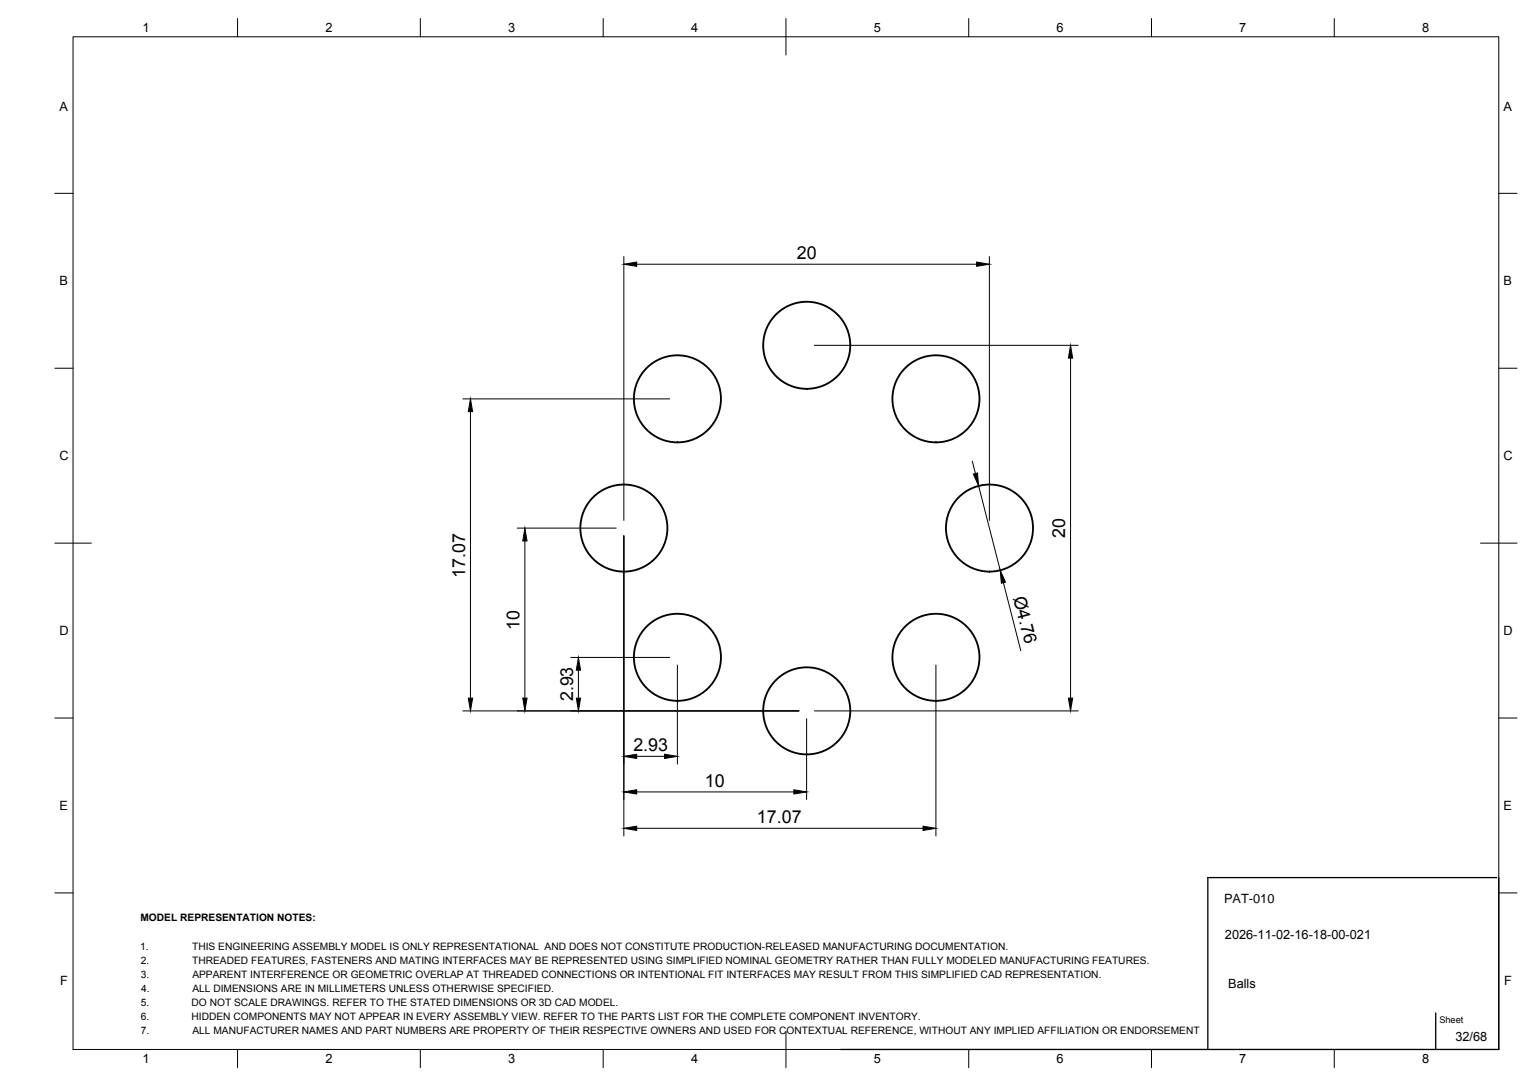
ISO-10303-21;
HEADER;
/* Generated by software containing ST-Developer
 * from STEP Tools, Inc. (www.steptools.com) 
 */

FILE_DESCRIPTION(
/* description */ ('Belt conveyor head drive unit'),
/* implementation_level */ '2;1');

FILE_NAME(
/* name */ 'Balls.step',
/* time_stamp */ '2026-10-28T03:26:19-07:00',
/* author */ (''),
/* organization */ (''),
/* preprocessor_version */ 'ST-DEVELOPER v20.2',
/* originating_system */ 'Autodesk Translation Framework v15.17.0.0',
/* authorisation */ '');

FILE_SCHEMA (('AUTOMOTIVE_DESIGN { 1 0 10303 214 3 1 1 }'));
ENDSEC;

DATA;
#10=MECHANICAL_DESIGN_GEOMETRIC_PRESENTATION_REPRESENTATION('',(#876,#877,#878,#879,#880,#881,#882,#883),#27069);
#645=SPHERICAL_SURFACE('',#15231,0.23815);
#646=SPHERICAL_SURFACE('',#15233,0.23815);
#647=SPHERICAL_SURFACE('',#15235,0.23815);
#648=SPHERICAL_SURFACE('',#15237,0.23815);
#649=SPHERICAL_SURFACE('',#15239,0.23815);
#650=SPHERICAL_SURFACE('',#15241,0.23815);
#651=SPHERICAL_SURFACE('',#15243,0.23815);
#652=SPHERICAL_SURFACE('',#15245,0.23815);
#738=SHAPE_REPRESENTATION_RELATIONSHIP('SRR','None',#27383,#807);
#807=ADVANCED_BREP_SHAPE_REPRESENTATION('',(#961,#962,#963,#964,#965,#966,
#967,#968),#27025);
#876=STYLED_ITEM('',(#27797),#961);
#877=STYLED_ITEM('',(#27797),#962);
#878=STYLED_ITEM('',(#27797),#963);
#879=STYLED_ITEM('',(#27797),#964);
#880=STYLED_ITEM('',(#27797),#965);
#881=STYLED_ITEM('',(#27797),#966);
#882=STYLED_ITEM('',(#27797),#967);
#883=STYLED_ITEM('',(#27797),#968);
#961=MANIFOLD_SOLID_BREP('Body1',#13741);
#962=MANIFOLD_SOLID_BREP('Body2',#13742);
#963=MANIFOLD_SOLID_BREP('Body3',#13743);
#964=MANIFOLD_SOLID_BREP('Body4',#13744);
#965=MANIFOLD_SOLID_BREP('Body5',#13745);
#966=MANIFOLD_SOLID_BREP('Body6',#13746);
#967=MANIFOLD_SOLID_BREP('Body7',#13747);
#968=MANIFOLD_SOLID_BREP('Body8',#13748);
#1951=FACE_OUTER_BOUND('',#2894,.T.);
#1952=FACE_OUTER_BOUND('',#2895,.T.);
#1953=FACE_OUTER_BOUND('',#2896,.T.);
#1954=FACE_OUTER_BOUND('',#2897,.T.);
#1955=FACE_OUTER_BOUND('',#2898,.T.);
#1956=FACE_OUTER_BOUND('',#2899,.T.);
#1957=FACE_OUTER_BOUND('',#2900,.T.);
#1958=FACE_OUTER_BOUND('',#2901,.T.);
#2894=EDGE_LOOP('',(#10336,#10337));
#2895=EDGE_LOOP('',(#10338,#10339));
#2896=EDGE_LOOP('',(#10340,#10341));
#2897=EDGE_LOOP('',(#10342,#10343));
#2898=EDGE_LOOP('',(#10344,#10345));
#2899=EDGE_LOOP('',(#10346,#10347));
#2900=EDGE_LOOP('',(#10348,#10349));
#2901=EDGE_LOOP('',(#10350,#10351));
#5400=CIRCLE('',#15232,0.23815);
#5401=CIRCLE('',#15234,0.23815);
#5402=CIRCLE('',#15236,0.23815);
#5403=CIRCLE('',#15238,0.23815);
#5404=CIRCLE('',#15240,0.23815);
#5405=CIRCLE('',#15242,0.23815);
#5406=CIRCLE('',#15244,0.23815);
#5407=CIRCLE('',#15246,0.23815);
#6411=VERTEX_POINT('',#22469);
#6412=VERTEX_POINT('',#22470);
#6413=VERTEX_POINT('',#22473);
#6414=VERTEX_POINT('',#22474);
#6415=VERTEX_POINT('',#22477);
#6416=VERTEX_POINT('',#22478);
#6417=VERTEX_POINT('',#22481);
#6418=VERTEX_POINT('',#22482);
#6419=VERTEX_POINT('',#22485);
#6420=VERTEX_POINT('',#22486);
#6421=VERTEX_POINT('',#22489);
#6422=VERTEX_POINT('',#22490);
#6423=VERTEX_POINT('',#22493);
#6424=VERTEX_POINT('',#22494);
#6425=VERTEX_POINT('',#22497);
#6426=VERTEX_POINT('',#22498);
#7860=EDGE_CURVE('',#6411,#6412,#5400,.T.);
#7861=EDGE_CURVE('',#6413,#6414,#5401,.T.);
#7862=EDGE_CURVE('',#6415,#6416,#5402,.T.);
#7863=EDGE_CURVE('',#6417,#6418,#5403,.T.);
#7864=EDGE_CURVE('',#6419,#6420,#5404,.T.);
#7865=EDGE_CURVE('',#6421,#6422,#5405,.T.);
#7866=EDGE_CURVE('',#6423,#6424,#5406,.T.);
#7867=EDGE_CURVE('',#6425,#6426,#5407,.T.);
#10336=ORIENTED_EDGE('',*,*,#7860,.T.);
#10337=ORIENTED_EDGE('',*,*,#7860,.F.);
#10338=ORIENTED_EDGE('',*,*,#7861,.T.);
#10339=ORIENTED_EDGE('',*,*,#7861,.F.);
#10340=ORIENTED_EDGE('',*,*,#7862,.T.);
#10341=ORIENTED_EDGE('',*,*,#7862,.F.);
#10342=ORIENTED_EDGE('',*,*,#7863,.T.);
#10343=ORIENTED_EDGE('',*,*,#7863,.F.);
#10344=ORIENTED_EDGE('',*,*,#7864,.T.);
#10345=ORIENTED_EDGE('',*,*,#7864,.F.);
#10346=ORIENTED_EDGE('',*,*,#7865,.T.);
#10347=ORIENTED_EDGE('',*,*,#7865,.F.);
#10348=ORIENTED_EDGE('',*,*,#7866,.T.);
#10349=ORIENTED_EDGE('',*,*,#7866,.F.);
#10350=ORIENTED_EDGE('',*,*,#7867,.T.);
#10351=ORIENTED_EDGE('',*,*,#7867,.F.);
#13230=ADVANCED_FACE('',(#1951),#645,.T.);
#13231=ADVANCED_FACE('',(#1952),#646,.T.);
#13232=ADVANCED_FACE('',(#1953),#647,.T.);
#13233=ADVANCED_FACE('',(#1954),#648,.T.);
#13234=ADVANCED_FACE('',(#1955),#649,.T.);
#13235=ADVANCED_FACE('',(#1956),#650,.T.);
#13236=ADVANCED_FACE('',(#1957),#651,.T.);
#13237=ADVANCED_FACE('',(#1958),#652,.T.);
#13741=CLOSED_SHELL('',(#13230));
#13742=CLOSED_SHELL('',(#13231));
#13743=CLOSED_SHELL('',(#13232));
#13744=CLOSED_SHELL('',(#13233));
#13745=CLOSED_SHELL('',(#13234));
#13746=CLOSED_SHELL('',(#13235));
#13747=CLOSED_SHELL('',(#13236));
#13748=CLOSED_SHELL('',(#13237));
#15230=AXIS2_PLACEMENT_3D('',#22467,#18141,#18142);
#15231=AXIS2_PLACEMENT_3D('',#22468,#18143,#18144);
#15232=AXIS2_PLACEMENT_3D('',#22471,#18145,#18146);
#15233=AXIS2_PLACEMENT_3D('',#22472,#18147,#18148);
#15234=AXIS2_PLACEMENT_3D('',#22475,#18149,#18150);
#15235=AXIS2_PLACEMENT_3D('',#22476,#18151,#18152);
#15236=AXIS2_PLACEMENT_3D('',#22479,#18153,#18154);
#15237=AXIS2_PLACEMENT_3D('',#22480,#18155,#18156);
#15238=AXIS2_PLACEMENT_3D('',#22483,#18157,#18158);
#15239=AXIS2_PLACEMENT_3D('',#22484,#18159,#18160);
#15240=AXIS2_PLACEMENT_3D('',#22487,#18161,#18162);
#15241=AXIS2_PLACEMENT_3D('',#22488,#18163,#18164);
#15242=AXIS2_PLACEMENT_3D('',#22491,#18165,#18166);
#15243=AXIS2_PLACEMENT_3D('',#22492,#18167,#18168);
#15244=AXIS2_PLACEMENT_3D('',#22495,#18169,#18170);
#15245=AXIS2_PLACEMENT_3D('',#22496,#18171,#18172);
#15246=AXIS2_PLACEMENT_3D('',#22499,#18173,#18174);
#18141=DIRECTION('axis',(0.,0.,1.));
#18142=DIRECTION('refdir',(1.,0.,0.));
#18143=DIRECTION('center_axis',(0.,0.,1.));
#18144=DIRECTION('ref_axis',(1.,0.,0.));
#18145=DIRECTION('center_axis',(1.22464679914735E-16,-1.,0.));
#18146=DIRECTION('ref_axis',(-1.,-1.22464679914735E-16,0.));
#18147=DIRECTION('center_axis',(0.707106781186548,0.,0.707106781186548));
#18148=DIRECTION('ref_axis',(0.707106781186548,0.,-0.707106781186548));
#18149=DIRECTION('center_axis',(8.65956056235494E-17,-1.,-8.65956056235493E-17));
#18150=DIRECTION('ref_axis',(-0.707106781186547,-1.22464679914735E-16,0.707106781186547));
#18151=DIRECTION('center_axis',(1.,0.,0.));
#18152=DIRECTION('ref_axis',(6.12323399573676E-17,0.,-1.));
#18153=DIRECTION('center_axis',(7.49879891330929E-33,-1.,-1.22464679914735E-16));
#18154=DIRECTION('ref_axis',(-6.12323399573676E-17,-1.22464679914735E-16,
1.));
#18155=DIRECTION('center_axis',(0.707106781186548,0.,-0.707106781186548));
#18156=DIRECTION('ref_axis',(-0.707106781186548,0.,-0.707106781186548));
#18157=DIRECTION('center_axis',(-8.65956056235493E-17,-1.,-8.65956056235494E-17));
#18158=DIRECTION('ref_axis',(0.707106781186547,-1.22464679914735E-16,0.707106781186547));
#18159=DIRECTION('center_axis',(0.,0.,-1.));
#18160=DIRECTION('ref_axis',(-1.,0.,-1.22464679914735E-16));
#18161=DIRECTION('center_axis',(-1.22464679914735E-16,-1.,-1.49975978266186E-32));
#18162=DIRECTION('ref_axis',(1.,-1.22464679914735E-16,1.22464679914735E-16));
#18163=DIRECTION('center_axis',(-0.707106781186547,0.,-0.707106781186548));
#18164=DIRECTION('ref_axis',(-0.707106781186548,0.,0.707106781186547));
#18165=DIRECTION('center_axis',(-8.65956056235493E-17,-1.,8.65956056235493E-17));
#18166=DIRECTION('ref_axis',(0.707106781186548,-1.22464679914735E-16,-0.707106781186547));
#18167=DIRECTION('center_axis',(-1.,0.,0.));
#18168=DIRECTION('ref_axis',(-1.83697019872103E-16,0.,1.));
#18169=DIRECTION('center_axis',(-2.24963967399279E-32,-1.,1.22464679914735E-16));
#18170=DIRECTION('ref_axis',(1.83697019872103E-16,-1.22464679914735E-16,
-1.));
#18171=DIRECTION('center_axis',(-0.707106781186548,0.,0.707106781186548));
#18172=DIRECTION('ref_axis',(0.707106781186547,0.,0.707106781186548));
#18173=DIRECTION('center_axis',(8.65956056235493E-17,-1.,8.65956056235493E-17));
#18174=DIRECTION('ref_axis',(-0.707106781186547,-1.22464679914735E-16,-0.707106781186548));
#22467=CARTESIAN_POINT('',(0.,0.,0.));
#22468=CARTESIAN_POINT('Origin',(1.,0.,0.));
#22469=CARTESIAN_POINT('',(1.,-1.78583896120461E-33,0.23815));
#22470=CARTESIAN_POINT('',(1.,-1.78583896120461E-33,-0.23815));
#22471=CARTESIAN_POINT('Origin',(1.,0.,0.));
#22472=CARTESIAN_POINT('Origin',(0.707106781186548,0.,-0.707106781186547));
#22473=CARTESIAN_POINT('',(0.875504261126124,-1.78583896120461E-33,-0.538709301246971));
#22474=CARTESIAN_POINT('',(0.538709301246971,-1.78583896120461E-33,-0.875504261126124));
#22475=CARTESIAN_POINT('Origin',(0.707106781186548,0.,-0.707106781186547));
#22476=CARTESIAN_POINT('Origin',(6.12323399573677E-17,0.,-1.));
#22477=CARTESIAN_POINT('',(0.23815,-1.78583896120461E-33,-1.));
#22478=CARTESIAN_POINT('',(-0.23815,-1.78583896120461E-33,-1.));
#22479=CARTESIAN_POINT('Origin',(6.12323399573677E-17,0.,-1.));
#22480=CARTESIAN_POINT('Origin',(-0.707106781186547,0.,-0.707106781186548));
#22481=CARTESIAN_POINT('',(-0.538709301246971,-1.78583896120461E-33,-0.875504261126124));
#22482=CARTESIAN_POINT('',(-0.875504261126124,-1.78583896120461E-33,-0.538709301246971));
#22483=CARTESIAN_POINT('Origin',(-0.707106781186547,0.,-0.707106781186548));
#22484=CARTESIAN_POINT('Origin',(-1.,0.,-1.22464679914735E-16));
#22485=CARTESIAN_POINT('',(-1.,-1.78583896120461E-33,-0.23815));
#22486=CARTESIAN_POINT('',(-1.,-1.78583896120461E-33,0.23815));
#22487=CARTESIAN_POINT('Origin',(-1.,0.,-1.22464679914735E-16));
#22488=CARTESIAN_POINT('Origin',(-0.707106781186548,0.,0.707106781186547));
#22489=CARTESIAN_POINT('',(-0.875504261126124,-7.94881478324376E-33,0.538709301246971));
#22490=CARTESIAN_POINT('',(-0.538709301246971,4.37713686083455E-33,0.875504261126124));
#22491=CARTESIAN_POINT('Origin',(-0.707106781186548,0.,0.707106781186547));
#22492=CARTESIAN_POINT('Origin',(-1.83697019872103E-16,0.,1.));
#22493=CARTESIAN_POINT('',(-0.23815,-1.78583896120461E-33,1.));
#22494=CARTESIAN_POINT('',(0.23815,-1.78583896120461E-33,1.));
#22495=CARTESIAN_POINT('Origin',(-1.83697019872103E-16,0.,1.));
#22496=CARTESIAN_POINT('Origin',(0.707106781186547,0.,0.707106781186548));
#22497=CARTESIAN_POINT('',(0.538709301246971,-4.86732687222419E-33,0.875504261126124));
#22498=CARTESIAN_POINT('',(0.875504261126124,1.29564894981497E-33,0.538709301246971));
#22499=CARTESIAN_POINT('Origin',(0.707106781186547,0.,0.707106781186548));
#26948=UNCERTAINTY_MEASURE_WITH_UNIT(LENGTH_MEASURE(0.001),#27070,
'DISTANCE_ACCURACY_VALUE',
'Maximum model space distance between geometric entities at asserted c
onnectivities');
#26992=UNCERTAINTY_MEASURE_WITH_UNIT(LENGTH_MEASURE(0.001),#27070,
'DISTANCE_ACCURACY_VALUE',
'Maximum model space distance between geometric entities at asserted c
onnectivities');
#27025=(
GEOMETRIC_REPRESENTATION_CONTEXT(3)
GLOBAL_UNCERTAINTY_ASSIGNED_CONTEXT((#26948))
GLOBAL_UNIT_ASSIGNED_CONTEXT((#27070,#27072,#27073))
REPRESENTATION_CONTEXT('','3D')
);
#27069=(
GEOMETRIC_REPRESENTATION_CONTEXT(3)
GLOBAL_UNCERTAINTY_ASSIGNED_CONTEXT((#26992))
GLOBAL_UNIT_ASSIGNED_CONTEXT((#27070,#27072,#27073))
REPRESENTATION_CONTEXT('','3D')
);
#27070=(
LENGTH_UNIT()
NAMED_UNIT(*)
SI_UNIT(.CENTI.,.METRE.)
);
#27072=(
NAMED_UNIT(*)
PLANE_ANGLE_UNIT()
SI_UNIT($,.RADIAN.)
);
#27073=(
NAMED_UNIT(*)
SI_UNIT($,.STERADIAN.)
SOLID_ANGLE_UNIT()
);
#27106=SHAPE_DEFINITION_REPRESENTATION(#27182,#27383);
#27182=PRODUCT_DEFINITION_SHAPE('',$,#27460);
#27383=SHAPE_REPRESENTATION('',(#15230),#27025);
#27427=PRODUCT_DEFINITION_CONTEXT('part definition',#27657,'design');
#27460=PRODUCT_DEFINITION('Balls','Balls',#27536,#27427);
#27536=PRODUCT_DEFINITION_FORMATION('',$,#27691);
#27657=APPLICATION_CONTEXT(
'Core Data for Automotive Mechanical Design Process');
#27658=PRODUCT_CONTEXT('part definition',#27657,'mechanical');
#27691=PRODUCT('Balls','Balls','Balls',(#27658));
#27791=COLOUR_RGB('Grey',0.48,0.52,0.57);
#27792=FILL_AREA_STYLE_COLOUR('',#27791);
#27793=FILL_AREA_STYLE('',(#27792));
#27794=SURFACE_STYLE_FILL_AREA(#27793);
#27795=SURFACE_SIDE_STYLE('',(#27794));
#27796=SURFACE_STYLE_USAGE(.BOTH.,#27795);
#27797=PRESENTATION_STYLE_ASSIGNMENT((#27796));
ENDSEC;
END-ISO-10303-21;
